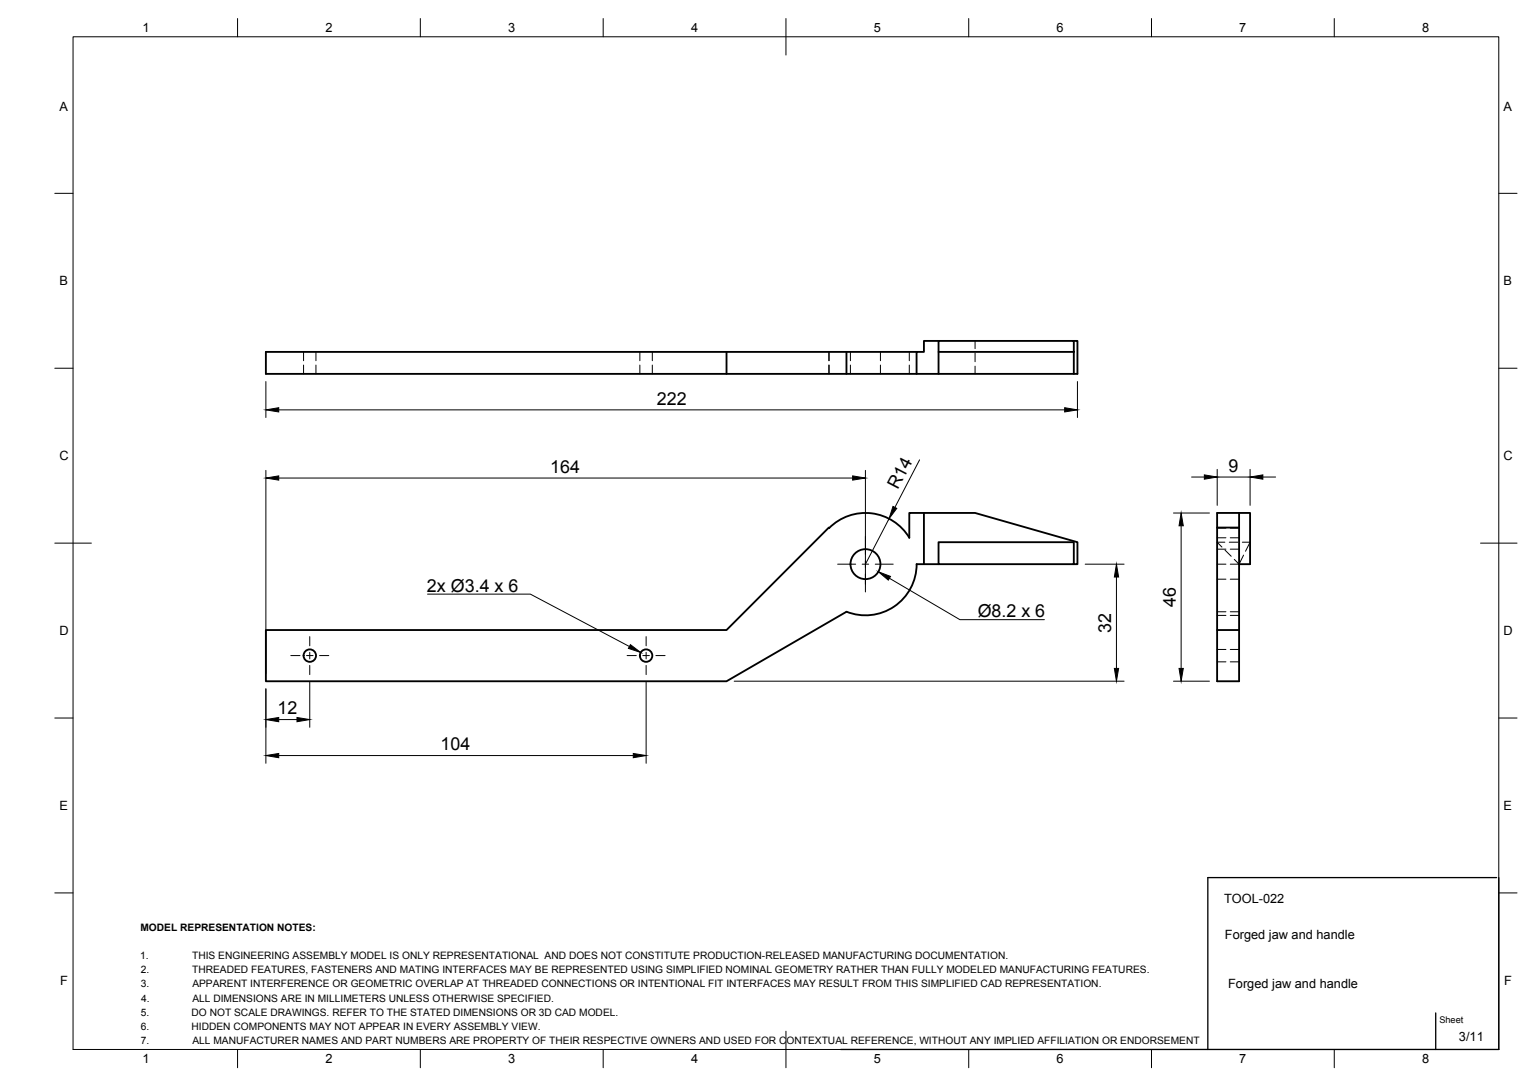
ISO-10303-21;
HEADER;
/* Generated by software containing ST-Developer
 * from STEP Tools, Inc. (www.steptools.com) 
 */

FILE_DESCRIPTION(
/* description */ (''),
/* implementation_level */ '2;1');

FILE_NAME(
/* name */ 'Forged jaw and handle.step',
/* time_stamp */ '2026-11-10T08:27:36-08:00',
/* author */ (''),
/* organization */ (''),
/* preprocessor_version */ 'ST-DEVELOPER v20.2',
/* originating_system */ 'Autodesk Translation Framework v15.17.0.0',
/* authorisation */ '');

FILE_SCHEMA (('AUTOMOTIVE_DESIGN { 1 0 10303 214 3 1 1 }'));
ENDSEC;

DATA;
#10=MECHANICAL_DESIGN_GEOMETRIC_PRESENTATION_REPRESENTATION('',(#566),#19090);
#546=SHAPE_REPRESENTATION_RELATIONSHIP('SRR','None',#19136,#556);
#556=ADVANCED_BREP_SHAPE_REPRESENTATION('',(#576),#19079);
#566=STYLED_ITEM('',(#19200),#576);
#576=MANIFOLD_SOLID_BREP('Body1',#6820);
#586=FACE_BOUND('',#1212,.T.);
#587=FACE_BOUND('',#1213,.T.);
#588=FACE_BOUND('',#1214,.T.);
#589=FACE_BOUND('',#1223,.T.);
#590=FACE_BOUND('',#1224,.T.);
#591=FACE_BOUND('',#1225,.T.);
#653=PLANE('',#6952);
#654=PLANE('',#6953);
#655=PLANE('',#6954);
#656=PLANE('',#6955);
#657=PLANE('',#6956);
#658=PLANE('',#6957);
#659=PLANE('',#6958);
#660=PLANE('',#6959);
#661=PLANE('',#6962);
#662=PLANE('',#6963);
#663=PLANE('',#6964);
#664=PLANE('',#6965);
#665=PLANE('',#6966);
#666=PLANE('',#6967);
#667=PLANE('',#6968);
#668=PLANE('',#6969);
#669=PLANE('',#6973);
#670=PLANE('',#6974);
#671=PLANE('',#6975);
#672=PLANE('',#6976);
#673=PLANE('',#6977);
#674=PLANE('',#6978);
#813=FACE_OUTER_BOUND('',#1201,.T.);
#814=FACE_OUTER_BOUND('',#1202,.T.);
#815=FACE_OUTER_BOUND('',#1203,.T.);
#816=FACE_OUTER_BOUND('',#1204,.T.);
#817=FACE_OUTER_BOUND('',#1205,.T.);
#818=FACE_OUTER_BOUND('',#1206,.T.);
#819=FACE_OUTER_BOUND('',#1207,.T.);
#820=FACE_OUTER_BOUND('',#1208,.T.);
#821=FACE_OUTER_BOUND('',#1209,.T.);
#822=FACE_OUTER_BOUND('',#1210,.T.);
#823=FACE_OUTER_BOUND('',#1211,.T.);
#824=FACE_OUTER_BOUND('',#1215,.T.);
#825=FACE_OUTER_BOUND('',#1216,.T.);
#826=FACE_OUTER_BOUND('',#1217,.T.);
#827=FACE_OUTER_BOUND('',#1218,.T.);
#828=FACE_OUTER_BOUND('',#1219,.T.);
#829=FACE_OUTER_BOUND('',#1220,.T.);
#830=FACE_OUTER_BOUND('',#1221,.T.);
#831=FACE_OUTER_BOUND('',#1222,.T.);
#832=FACE_OUTER_BOUND('',#1226,.T.);
#833=FACE_OUTER_BOUND('',#1227,.T.);
#834=FACE_OUTER_BOUND('',#1228,.T.);
#835=FACE_OUTER_BOUND('',#1229,.T.);
#836=FACE_OUTER_BOUND('',#1230,.T.);
#837=FACE_OUTER_BOUND('',#1231,.T.);
#838=FACE_OUTER_BOUND('',#1232,.T.);
#839=FACE_OUTER_BOUND('',#1233,.T.);
#1201=EDGE_LOOP('',(#4335,#4336,#4337,#4338));
#1202=EDGE_LOOP('',(#4339,#4340,#4341,#4342));
#1203=EDGE_LOOP('',(#4343,#4344,#4345,#4346));
#1204=EDGE_LOOP('',(#4347,#4348,#4349));
#1205=EDGE_LOOP('',(#4350,#4351,#4352,#4353));
#1206=EDGE_LOOP('',(#4354,#4355,#4356));
#1207=EDGE_LOOP('',(#4357,#4358,#4359,#4360,#4361,#4362,#4363));
#1208=EDGE_LOOP('',(#4364,#4365,#4366));
#1209=EDGE_LOOP('',(#4367,#4368,#4369,#4370));
#1210=EDGE_LOOP('',(#4371,#4372,#4373));
#1211=EDGE_LOOP('',(#4374,#4375,#4376,#4377,#4378,#4379,#4380,#4381,#4382,
#4383,#4384,#4385,#4386,#4387,#4388,#4389,#4390));
#1212=EDGE_LOOP('',(#4391));
#1213=EDGE_LOOP('',(#4392));
#1214=EDGE_LOOP('',(#4393));
#1215=EDGE_LOOP('',(#4394,#4395,#4396,#4397));
#1216=EDGE_LOOP('',(#4398,#4399,#4400,#4401,#4402,#4403,#4404,#4405,#4406));
#1217=EDGE_LOOP('',(#4407,#4408,#4409,#4410,#4411));
#1218=EDGE_LOOP('',(#4412,#4413,#4414,#4415));
#1219=EDGE_LOOP('',(#4416,#4417,#4418,#4419));
#1220=EDGE_LOOP('',(#4420,#4421,#4422,#4423));
#1221=EDGE_LOOP('',(#4424,#4425,#4426,#4427,#4428,#4429));
#1222=EDGE_LOOP('',(#4430,#4431,#4432,#4433,#4434,#4435,#4436,#4437,#4438,
#4439,#4440,#4441));
#1223=EDGE_LOOP('',(#4442));
#1224=EDGE_LOOP('',(#4443));
#1225=EDGE_LOOP('',(#4444));
#1226=EDGE_LOOP('',(#4445,#4446,#4447,#4448));
#1227=EDGE_LOOP('',(#4449,#4450,#4451,#4452));
#1228=EDGE_LOOP('',(#4453,#4454,#4455,#4456));
#1229=EDGE_LOOP('',(#4457,#4458,#4459,#4460));
#1230=EDGE_LOOP('',(#4461,#4462,#4463,#4464));
#1231=EDGE_LOOP('',(#4465,#4466,#4467,#4468));
#1232=EDGE_LOOP('',(#4469,#4470,#4471,#4472));
#1233=EDGE_LOOP('',(#4473,#4474,#4475,#4476));
#1656=LINE('',#8884,#2105);
#1657=LINE('',#8890,#2106);
#1658=LINE('',#8896,#2107);
#1659=LINE('',#8901,#2108);
#1660=LINE('',#8903,#2109);
#1661=LINE('',#8904,#2110);
#1662=LINE('',#8908,#2111);
#1663=LINE('',#8909,#2112);
#1664=LINE('',#8910,#2113);
#1665=LINE('',#8913,#2114);
#1666=LINE('',#8914,#2115);
#1667=LINE('',#8917,#2116);
#1668=LINE('',#8919,#2117);
#1669=LINE('',#8921,#2118);
#1670=LINE('',#8923,#2119);
#1671=LINE('',#8925,#2120);
#1672=LINE('',#8926,#2121);
#1673=LINE('',#8929,#2122);
#1674=LINE('',#8930,#2123);
#1675=LINE('',#8933,#2124);
#1676=LINE('',#8934,#2125);
#1677=LINE('',#8937,#2126);
#1678=LINE('',#8938,#2127);
#1679=LINE('',#8943,#2128);
#1680=LINE('',#8945,#2129);
#1681=LINE('',#8947,#2130);
#1682=LINE('',#8949,#2131);
#1683=LINE('',#8951,#2132);
#1684=LINE('',#8953,#2133);
#1685=LINE('',#8957,#2134);
#1686=LINE('',#8959,#2135);
#1687=LINE('',#8961,#2136);
#1688=LINE('',#8963,#2137);
#1689=LINE('',#8964,#2138);
#1690=LINE('',#8967,#2139);
#1691=LINE('',#8969,#2140);
#1692=LINE('',#8970,#2141);
#1693=LINE('',#8973,#2142);
#1694=LINE('',#8975,#2143);
#1695=LINE('',#8977,#2144);
#1696=LINE('',#8978,#2145);
#1697=LINE('',#8980,#2146);
#1698=LINE('',#8983,#2147);
#1699=LINE('',#8985,#2148);
#1700=LINE('',#8986,#2149);
#1701=LINE('',#8988,#2150);
#1702=LINE('',#8990,#2151);
#1703=LINE('',#8992,#2152);
#1704=LINE('',#8997,#2153);
#1705=LINE('',#8999,#2154);
#1706=LINE('',#9001,#2155);
#1707=LINE('',#9003,#2156);
#1708=LINE('',#9005,#2157);
#1709=LINE('',#9007,#2158);
#1710=LINE('',#9010,#2159);
#1711=LINE('',#9012,#2160);
#1712=LINE('',#9013,#2161);
#1713=LINE('',#9015,#2162);
#1714=LINE('',#9017,#2163);
#1715=LINE('',#9019,#2164);
#1716=LINE('',#9021,#2165);
#2105=VECTOR('',#7445,0.17);
#2106=VECTOR('',#7452,0.17);
#2107=VECTOR('',#7459,0.41);
#2108=VECTOR('',#7464,1.);
#2109=VECTOR('',#7465,1.);
#2110=VECTOR('',#7466,1.);
#2111=VECTOR('',#7469,1.);
#2112=VECTOR('',#7470,1.);
#2113=VECTOR('',#7471,1.);
#2114=VECTOR('',#7474,1.);
#2115=VECTOR('',#7475,1.);
#2116=VECTOR('',#7478,1.);
#2117=VECTOR('',#7479,1.);
#2118=VECTOR('',#7480,1.);
#2119=VECTOR('',#7481,1.);
#2120=VECTOR('',#7482,1.);
#2121=VECTOR('',#7483,1.);
#2122=VECTOR('',#7486,1.);
#2123=VECTOR('',#7487,1.);
#2124=VECTOR('',#7490,1.);
#2125=VECTOR('',#7491,1.);
#2126=VECTOR('',#7494,1.);
#2127=VECTOR('',#7495,1.);
#2128=VECTOR('',#7500,1.);
#2129=VECTOR('',#7501,1.);
#2130=VECTOR('',#7502,1.);
#2131=VECTOR('',#7503,1.);
#2132=VECTOR('',#7504,1.);
#2133=VECTOR('',#7505,1.);
#2134=VECTOR('',#7508,1.);
#2135=VECTOR('',#7509,1.);
#2136=VECTOR('',#7510,1.);
#2137=VECTOR('',#7511,1.);
#2138=VECTOR('',#7512,1.);
#2139=VECTOR('',#7515,1.);
#2140=VECTOR('',#7516,1.);
#2141=VECTOR('',#7517,1.);
#2142=VECTOR('',#7520,1.);
#2143=VECTOR('',#7521,1.);
#2144=VECTOR('',#7522,1.);
#2145=VECTOR('',#7523,1.);
#2146=VECTOR('',#7526,1.);
#2147=VECTOR('',#7529,1.);
#2148=VECTOR('',#7530,1.);
#2149=VECTOR('',#7531,1.);
#2150=VECTOR('',#7534,1.);
#2151=VECTOR('',#7537,1.);
#2152=VECTOR('',#7540,1.);
#2153=VECTOR('',#7545,1.);
#2154=VECTOR('',#7546,1.);
#2155=VECTOR('',#7547,1.);
#2156=VECTOR('',#7548,1.);
#2157=VECTOR('',#7549,1.);
#2158=VECTOR('',#7550,1.);
#2159=VECTOR('',#7555,1.);
#2160=VECTOR('',#7558,1.);
#2161=VECTOR('',#7559,1.);
#2162=VECTOR('',#7562,1.);
#2163=VECTOR('',#7565,1.);
#2164=VECTOR('',#7568,1.);
#2165=VECTOR('',#7571,1.);
#2554=CIRCLE('',#6944,0.17);
#2555=CIRCLE('',#6945,0.17);
#2556=CIRCLE('',#6947,0.17);
#2557=CIRCLE('',#6948,0.17);
#2558=CIRCLE('',#6950,0.41);
#2559=CIRCLE('',#6951,0.41);
#2560=CIRCLE('',#6960,1.4);
#2561=CIRCLE('',#6961,1.4);
#2562=CIRCLE('',#6970,1.4);
#2563=CIRCLE('',#6971,1.4);
#2714=VERTEX_POINT('',#8881);
#2715=VERTEX_POINT('',#8883);
#2716=VERTEX_POINT('',#8887);
#2717=VERTEX_POINT('',#8889);
#2718=VERTEX_POINT('',#8893);
#2719=VERTEX_POINT('',#8895);
#2720=VERTEX_POINT('',#8899);
#2721=VERTEX_POINT('',#8900);
#2722=VERTEX_POINT('',#8902);
#2723=VERTEX_POINT('',#8906);
#2724=VERTEX_POINT('',#8907);
#2725=VERTEX_POINT('',#8912);
#2726=VERTEX_POINT('',#8916);
#2727=VERTEX_POINT('',#8918);
#2728=VERTEX_POINT('',#8920);
#2729=VERTEX_POINT('',#8922);
#2730=VERTEX_POINT('',#8924);
#2731=VERTEX_POINT('',#8928);
#2732=VERTEX_POINT('',#8932);
#2733=VERTEX_POINT('',#8936);
#2734=VERTEX_POINT('',#8940);
#2735=VERTEX_POINT('',#8942);
#2736=VERTEX_POINT('',#8944);
#2737=VERTEX_POINT('',#8946);
#2738=VERTEX_POINT('',#8948);
#2739=VERTEX_POINT('',#8950);
#2740=VERTEX_POINT('',#8952);
#2741=VERTEX_POINT('',#8954);
#2742=VERTEX_POINT('',#8956);
#2743=VERTEX_POINT('',#8958);
#2744=VERTEX_POINT('',#8960);
#2745=VERTEX_POINT('',#8962);
#2746=VERTEX_POINT('',#8966);
#2747=VERTEX_POINT('',#8968);
#2748=VERTEX_POINT('',#8972);
#2749=VERTEX_POINT('',#8974);
#2750=VERTEX_POINT('',#8976);
#2751=VERTEX_POINT('',#8982);
#2752=VERTEX_POINT('',#8984);
#2753=VERTEX_POINT('',#8994);
#2754=VERTEX_POINT('',#8996);
#2755=VERTEX_POINT('',#8998);
#2756=VERTEX_POINT('',#9000);
#2757=VERTEX_POINT('',#9002);
#2758=VERTEX_POINT('',#9004);
#2759=VERTEX_POINT('',#9006);
#3352=EDGE_CURVE('',#2714,#2714,#2554,.T.);
#3353=EDGE_CURVE('',#2714,#2715,#1656,.T.);
#3354=EDGE_CURVE('',#2715,#2715,#2555,.T.);
#3355=EDGE_CURVE('',#2716,#2716,#2556,.T.);
#3356=EDGE_CURVE('',#2716,#2717,#1657,.T.);
#3357=EDGE_CURVE('',#2717,#2717,#2557,.T.);
#3358=EDGE_CURVE('',#2718,#2718,#2558,.T.);
#3359=EDGE_CURVE('',#2718,#2719,#1658,.T.);
#3360=EDGE_CURVE('',#2719,#2719,#2559,.T.);
#3361=EDGE_CURVE('',#2720,#2721,#1659,.T.);
#3362=EDGE_CURVE('',#2722,#2720,#1660,.T.);
#3363=EDGE_CURVE('',#2721,#2722,#1661,.T.);
#3364=EDGE_CURVE('',#2723,#2724,#1662,.T.);
#3365=EDGE_CURVE('',#2722,#2723,#1663,.T.);
#3366=EDGE_CURVE('',#2720,#2724,#1664,.T.);
#3367=EDGE_CURVE('',#2725,#2724,#1665,.T.);
#3368=EDGE_CURVE('',#2723,#2725,#1666,.T.);
#3369=EDGE_CURVE('',#2726,#2721,#1667,.T.);
#3370=EDGE_CURVE('',#2726,#2727,#1668,.T.);
#3371=EDGE_CURVE('',#2728,#2727,#1669,.T.);
#3372=EDGE_CURVE('',#2729,#2728,#1670,.T.);
#3373=EDGE_CURVE('',#2730,#2729,#1671,.T.);
#3374=EDGE_CURVE('',#2730,#2720,#1672,.T.);
#3375=EDGE_CURVE('',#2731,#2730,#1673,.T.);
#3376=EDGE_CURVE('',#2720,#2731,#1674,.T.);
#3377=EDGE_CURVE('',#2724,#2732,#1675,.T.);
#3378=EDGE_CURVE('',#2732,#2731,#1676,.T.);
#3379=EDGE_CURVE('',#2733,#2732,#1677,.T.);
#3380=EDGE_CURVE('',#2724,#2733,#1678,.T.);
#3381=EDGE_CURVE('',#2729,#2734,#2560,.T.);
#3382=EDGE_CURVE('',#2734,#2735,#1679,.T.);
#3383=EDGE_CURVE('',#2735,#2736,#1680,.T.);
#3384=EDGE_CURVE('',#2736,#2737,#1681,.T.);
#3385=EDGE_CURVE('',#2737,#2738,#1682,.T.);
#3386=EDGE_CURVE('',#2738,#2739,#1683,.T.);
#3387=EDGE_CURVE('',#2739,#2740,#1684,.T.);
#3388=EDGE_CURVE('',#2740,#2741,#2561,.T.);
#3389=EDGE_CURVE('',#2741,#2742,#1685,.T.);
#3390=EDGE_CURVE('',#2742,#2743,#1686,.T.);
#3391=EDGE_CURVE('',#2743,#2744,#1687,.T.);
#3392=EDGE_CURVE('',#2744,#2745,#1688,.T.);
#3393=EDGE_CURVE('',#2745,#2733,#1689,.T.);
#3394=EDGE_CURVE('',#2746,#2726,#1690,.T.);
#3395=EDGE_CURVE('',#2746,#2747,#1691,.T.);
#3396=EDGE_CURVE('',#2727,#2747,#1692,.T.);
#3397=EDGE_CURVE('',#2725,#2748,#1693,.T.);
#3398=EDGE_CURVE('',#2748,#2749,#1694,.T.);
#3399=EDGE_CURVE('',#2749,#2750,#1695,.T.);
#3400=EDGE_CURVE('',#2750,#2746,#1696,.T.);
#3401=EDGE_CURVE('',#2748,#2745,#1697,.T.);
#3402=EDGE_CURVE('',#2751,#2741,#1698,.T.);
#3403=EDGE_CURVE('',#2752,#2751,#1699,.T.);
#3404=EDGE_CURVE('',#2752,#2742,#1700,.T.);
#3405=EDGE_CURVE('',#2749,#2744,#1701,.T.);
#3406=EDGE_CURVE('',#2750,#2743,#1702,.T.);
#3407=EDGE_CURVE('',#2747,#2752,#1703,.T.);
#3408=EDGE_CURVE('',#2753,#2751,#2562,.T.);
#3409=EDGE_CURVE('',#2754,#2753,#1704,.T.);
#3410=EDGE_CURVE('',#2755,#2754,#1705,.T.);
#3411=EDGE_CURVE('',#2756,#2755,#1706,.T.);
#3412=EDGE_CURVE('',#2757,#2756,#1707,.T.);
#3413=EDGE_CURVE('',#2758,#2757,#1708,.T.);
#3414=EDGE_CURVE('',#2759,#2758,#1709,.T.);
#3415=EDGE_CURVE('',#2728,#2759,#2563,.T.);
#3416=EDGE_CURVE('',#2740,#2753,#1710,.T.);
#3417=EDGE_CURVE('',#2759,#2734,#1711,.T.);
#3418=EDGE_CURVE('',#2758,#2735,#1712,.T.);
#3419=EDGE_CURVE('',#2754,#2739,#1713,.T.);
#3420=EDGE_CURVE('',#2755,#2738,#1714,.T.);
#3421=EDGE_CURVE('',#2756,#2737,#1715,.T.);
#3422=EDGE_CURVE('',#2757,#2736,#1716,.T.);
#4335=ORIENTED_EDGE('',*,*,#3352,.F.);
#4336=ORIENTED_EDGE('',*,*,#3353,.T.);
#4337=ORIENTED_EDGE('',*,*,#3354,.F.);
#4338=ORIENTED_EDGE('',*,*,#3353,.F.);
#4339=ORIENTED_EDGE('',*,*,#3355,.F.);
#4340=ORIENTED_EDGE('',*,*,#3356,.T.);
#4341=ORIENTED_EDGE('',*,*,#3357,.F.);
#4342=ORIENTED_EDGE('',*,*,#3356,.F.);
#4343=ORIENTED_EDGE('',*,*,#3358,.F.);
#4344=ORIENTED_EDGE('',*,*,#3359,.T.);
#4345=ORIENTED_EDGE('',*,*,#3360,.F.);
#4346=ORIENTED_EDGE('',*,*,#3359,.F.);
#4347=ORIENTED_EDGE('',*,*,#3361,.F.);
#4348=ORIENTED_EDGE('',*,*,#3362,.F.);
#4349=ORIENTED_EDGE('',*,*,#3363,.F.);
#4350=ORIENTED_EDGE('',*,*,#3364,.F.);
#4351=ORIENTED_EDGE('',*,*,#3365,.F.);
#4352=ORIENTED_EDGE('',*,*,#3362,.T.);
#4353=ORIENTED_EDGE('',*,*,#3366,.T.);
#4354=ORIENTED_EDGE('',*,*,#3367,.F.);
#4355=ORIENTED_EDGE('',*,*,#3368,.F.);
#4356=ORIENTED_EDGE('',*,*,#3364,.T.);
#4357=ORIENTED_EDGE('',*,*,#3361,.T.);
#4358=ORIENTED_EDGE('',*,*,#3369,.F.);
#4359=ORIENTED_EDGE('',*,*,#3370,.T.);
#4360=ORIENTED_EDGE('',*,*,#3371,.F.);
#4361=ORIENTED_EDGE('',*,*,#3372,.F.);
#4362=ORIENTED_EDGE('',*,*,#3373,.F.);
#4363=ORIENTED_EDGE('',*,*,#3374,.T.);
#4364=ORIENTED_EDGE('',*,*,#3375,.F.);
#4365=ORIENTED_EDGE('',*,*,#3376,.F.);
#4366=ORIENTED_EDGE('',*,*,#3374,.F.);
#4367=ORIENTED_EDGE('',*,*,#3377,.F.);
#4368=ORIENTED_EDGE('',*,*,#3366,.F.);
#4369=ORIENTED_EDGE('',*,*,#3376,.T.);
#4370=ORIENTED_EDGE('',*,*,#3378,.F.);
#4371=ORIENTED_EDGE('',*,*,#3379,.F.);
#4372=ORIENTED_EDGE('',*,*,#3380,.F.);
#4373=ORIENTED_EDGE('',*,*,#3377,.T.);
#4374=ORIENTED_EDGE('',*,*,#3379,.T.);
#4375=ORIENTED_EDGE('',*,*,#3378,.T.);
#4376=ORIENTED_EDGE('',*,*,#3375,.T.);
#4377=ORIENTED_EDGE('',*,*,#3373,.T.);
#4378=ORIENTED_EDGE('',*,*,#3381,.T.);
#4379=ORIENTED_EDGE('',*,*,#3382,.T.);
#4380=ORIENTED_EDGE('',*,*,#3383,.T.);
#4381=ORIENTED_EDGE('',*,*,#3384,.T.);
#4382=ORIENTED_EDGE('',*,*,#3385,.T.);
#4383=ORIENTED_EDGE('',*,*,#3386,.T.);
#4384=ORIENTED_EDGE('',*,*,#3387,.T.);
#4385=ORIENTED_EDGE('',*,*,#3388,.T.);
#4386=ORIENTED_EDGE('',*,*,#3389,.T.);
#4387=ORIENTED_EDGE('',*,*,#3390,.T.);
#4388=ORIENTED_EDGE('',*,*,#3391,.T.);
#4389=ORIENTED_EDGE('',*,*,#3392,.T.);
#4390=ORIENTED_EDGE('',*,*,#3393,.T.);
#4391=ORIENTED_EDGE('',*,*,#3352,.T.);
#4392=ORIENTED_EDGE('',*,*,#3355,.T.);
#4393=ORIENTED_EDGE('',*,*,#3358,.T.);
#4394=ORIENTED_EDGE('',*,*,#3394,.F.);
#4395=ORIENTED_EDGE('',*,*,#3395,.T.);
#4396=ORIENTED_EDGE('',*,*,#3396,.F.);
#4397=ORIENTED_EDGE('',*,*,#3370,.F.);
#4398=ORIENTED_EDGE('',*,*,#3368,.T.);
#4399=ORIENTED_EDGE('',*,*,#3397,.T.);
#4400=ORIENTED_EDGE('',*,*,#3398,.T.);
#4401=ORIENTED_EDGE('',*,*,#3399,.T.);
#4402=ORIENTED_EDGE('',*,*,#3400,.T.);
#4403=ORIENTED_EDGE('',*,*,#3394,.T.);
#4404=ORIENTED_EDGE('',*,*,#3369,.T.);
#4405=ORIENTED_EDGE('',*,*,#3363,.T.);
#4406=ORIENTED_EDGE('',*,*,#3365,.T.);
#4407=ORIENTED_EDGE('',*,*,#3367,.T.);
#4408=ORIENTED_EDGE('',*,*,#3380,.T.);
#4409=ORIENTED_EDGE('',*,*,#3393,.F.);
#4410=ORIENTED_EDGE('',*,*,#3401,.F.);
#4411=ORIENTED_EDGE('',*,*,#3397,.F.);
#4412=ORIENTED_EDGE('',*,*,#3402,.F.);
#4413=ORIENTED_EDGE('',*,*,#3403,.F.);
#4414=ORIENTED_EDGE('',*,*,#3404,.T.);
#4415=ORIENTED_EDGE('',*,*,#3389,.F.);
#4416=ORIENTED_EDGE('',*,*,#3401,.T.);
#4417=ORIENTED_EDGE('',*,*,#3392,.F.);
#4418=ORIENTED_EDGE('',*,*,#3405,.F.);
#4419=ORIENTED_EDGE('',*,*,#3398,.F.);
#4420=ORIENTED_EDGE('',*,*,#3405,.T.);
#4421=ORIENTED_EDGE('',*,*,#3391,.F.);
#4422=ORIENTED_EDGE('',*,*,#3406,.F.);
#4423=ORIENTED_EDGE('',*,*,#3399,.F.);
#4424=ORIENTED_EDGE('',*,*,#3406,.T.);
#4425=ORIENTED_EDGE('',*,*,#3390,.F.);
#4426=ORIENTED_EDGE('',*,*,#3404,.F.);
#4427=ORIENTED_EDGE('',*,*,#3407,.F.);
#4428=ORIENTED_EDGE('',*,*,#3395,.F.);
#4429=ORIENTED_EDGE('',*,*,#3400,.F.);
#4430=ORIENTED_EDGE('',*,*,#3396,.T.);
#4431=ORIENTED_EDGE('',*,*,#3407,.T.);
#4432=ORIENTED_EDGE('',*,*,#3403,.T.);
#4433=ORIENTED_EDGE('',*,*,#3408,.F.);
#4434=ORIENTED_EDGE('',*,*,#3409,.F.);
#4435=ORIENTED_EDGE('',*,*,#3410,.F.);
#4436=ORIENTED_EDGE('',*,*,#3411,.F.);
#4437=ORIENTED_EDGE('',*,*,#3412,.F.);
#4438=ORIENTED_EDGE('',*,*,#3413,.F.);
#4439=ORIENTED_EDGE('',*,*,#3414,.F.);
#4440=ORIENTED_EDGE('',*,*,#3415,.F.);
#4441=ORIENTED_EDGE('',*,*,#3371,.T.);
#4442=ORIENTED_EDGE('',*,*,#3354,.T.);
#4443=ORIENTED_EDGE('',*,*,#3357,.T.);
#4444=ORIENTED_EDGE('',*,*,#3360,.T.);
#4445=ORIENTED_EDGE('',*,*,#3402,.T.);
#4446=ORIENTED_EDGE('',*,*,#3388,.F.);
#4447=ORIENTED_EDGE('',*,*,#3416,.T.);
#4448=ORIENTED_EDGE('',*,*,#3408,.T.);
#4449=ORIENTED_EDGE('',*,*,#3417,.F.);
#4450=ORIENTED_EDGE('',*,*,#3414,.T.);
#4451=ORIENTED_EDGE('',*,*,#3418,.T.);
#4452=ORIENTED_EDGE('',*,*,#3382,.F.);
#4453=ORIENTED_EDGE('',*,*,#3416,.F.);
#4454=ORIENTED_EDGE('',*,*,#3387,.F.);
#4455=ORIENTED_EDGE('',*,*,#3419,.F.);
#4456=ORIENTED_EDGE('',*,*,#3409,.T.);
#4457=ORIENTED_EDGE('',*,*,#3410,.T.);
#4458=ORIENTED_EDGE('',*,*,#3419,.T.);
#4459=ORIENTED_EDGE('',*,*,#3386,.F.);
#4460=ORIENTED_EDGE('',*,*,#3420,.F.);
#4461=ORIENTED_EDGE('',*,*,#3411,.T.);
#4462=ORIENTED_EDGE('',*,*,#3420,.T.);
#4463=ORIENTED_EDGE('',*,*,#3385,.F.);
#4464=ORIENTED_EDGE('',*,*,#3421,.F.);
#4465=ORIENTED_EDGE('',*,*,#3412,.T.);
#4466=ORIENTED_EDGE('',*,*,#3421,.T.);
#4467=ORIENTED_EDGE('',*,*,#3384,.F.);
#4468=ORIENTED_EDGE('',*,*,#3422,.F.);
#4469=ORIENTED_EDGE('',*,*,#3413,.T.);
#4470=ORIENTED_EDGE('',*,*,#3422,.T.);
#4471=ORIENTED_EDGE('',*,*,#3383,.F.);
#4472=ORIENTED_EDGE('',*,*,#3418,.F.);
#4473=ORIENTED_EDGE('',*,*,#3372,.T.);
#4474=ORIENTED_EDGE('',*,*,#3415,.T.);
#4475=ORIENTED_EDGE('',*,*,#3417,.T.);
#4476=ORIENTED_EDGE('',*,*,#3381,.F.);
#6301=CYLINDRICAL_SURFACE('',#6943,0.17);
#6302=CYLINDRICAL_SURFACE('',#6946,0.17);
#6303=CYLINDRICAL_SURFACE('',#6949,0.41);
#6304=CYLINDRICAL_SURFACE('',#6972,1.4);
#6305=CYLINDRICAL_SURFACE('',#6979,1.4);
#6432=ADVANCED_FACE('',(#813),#6301,.F.);
#6433=ADVANCED_FACE('',(#814),#6302,.F.);
#6434=ADVANCED_FACE('',(#815),#6303,.F.);
#6435=ADVANCED_FACE('',(#816),#653,.F.);
#6436=ADVANCED_FACE('',(#817),#654,.F.);
#6437=ADVANCED_FACE('',(#818),#655,.T.);
#6438=ADVANCED_FACE('',(#819),#656,.T.);
#6439=ADVANCED_FACE('',(#820),#657,.F.);
#6440=ADVANCED_FACE('',(#821),#658,.F.);
#6441=ADVANCED_FACE('',(#822),#659,.T.);
#6442=ADVANCED_FACE('',(#823,#586,#587,#588),#660,.T.);
#6443=ADVANCED_FACE('',(#824),#661,.T.);
#6444=ADVANCED_FACE('',(#825),#662,.F.);
#6445=ADVANCED_FACE('',(#826),#663,.T.);
#6446=ADVANCED_FACE('',(#827),#664,.T.);
#6447=ADVANCED_FACE('',(#828),#665,.T.);
#6448=ADVANCED_FACE('',(#829),#666,.T.);
#6449=ADVANCED_FACE('',(#830),#667,.T.);
#6450=ADVANCED_FACE('',(#831,#589,#590,#591),#668,.F.);
#6451=ADVANCED_FACE('',(#832),#6304,.T.);
#6452=ADVANCED_FACE('',(#833),#669,.T.);
#6453=ADVANCED_FACE('',(#834),#670,.T.);
#6454=ADVANCED_FACE('',(#835),#671,.T.);
#6455=ADVANCED_FACE('',(#836),#672,.T.);
#6456=ADVANCED_FACE('',(#837),#673,.T.);
#6457=ADVANCED_FACE('',(#838),#674,.T.);
#6458=ADVANCED_FACE('',(#839),#6305,.T.);
#6820=CLOSED_SHELL('',(#6432,#6433,#6434,#6435,#6436,#6437,#6438,#6439,
#6440,#6441,#6442,#6443,#6444,#6445,#6446,#6447,#6448,#6449,#6450,#6451,
#6452,#6453,#6454,#6455,#6456,#6457,#6458));
#6942=AXIS2_PLACEMENT_3D('',#8879,#7439,#7440);
#6943=AXIS2_PLACEMENT_3D('',#8880,#7441,#7442);
#6944=AXIS2_PLACEMENT_3D('',#8882,#7443,#7444);
#6945=AXIS2_PLACEMENT_3D('',#8885,#7446,#7447);
#6946=AXIS2_PLACEMENT_3D('',#8886,#7448,#7449);
#6947=AXIS2_PLACEMENT_3D('',#8888,#7450,#7451);
#6948=AXIS2_PLACEMENT_3D('',#8891,#7453,#7454);
#6949=AXIS2_PLACEMENT_3D('',#8892,#7455,#7456);
#6950=AXIS2_PLACEMENT_3D('',#8894,#7457,#7458);
#6951=AXIS2_PLACEMENT_3D('',#8897,#7460,#7461);
#6952=AXIS2_PLACEMENT_3D('',#8898,#7462,#7463);
#6953=AXIS2_PLACEMENT_3D('',#8905,#7467,#7468);
#6954=AXIS2_PLACEMENT_3D('',#8911,#7472,#7473);
#6955=AXIS2_PLACEMENT_3D('',#8915,#7476,#7477);
#6956=AXIS2_PLACEMENT_3D('',#8927,#7484,#7485);
#6957=AXIS2_PLACEMENT_3D('',#8931,#7488,#7489);
#6958=AXIS2_PLACEMENT_3D('',#8935,#7492,#7493);
#6959=AXIS2_PLACEMENT_3D('',#8939,#7496,#7497);
#6960=AXIS2_PLACEMENT_3D('',#8941,#7498,#7499);
#6961=AXIS2_PLACEMENT_3D('',#8955,#7506,#7507);
#6962=AXIS2_PLACEMENT_3D('',#8965,#7513,#7514);
#6963=AXIS2_PLACEMENT_3D('',#8971,#7518,#7519);
#6964=AXIS2_PLACEMENT_3D('',#8979,#7524,#7525);
#6965=AXIS2_PLACEMENT_3D('',#8981,#7527,#7528);
#6966=AXIS2_PLACEMENT_3D('',#8987,#7532,#7533);
#6967=AXIS2_PLACEMENT_3D('',#8989,#7535,#7536);
#6968=AXIS2_PLACEMENT_3D('',#8991,#7538,#7539);
#6969=AXIS2_PLACEMENT_3D('',#8993,#7541,#7542);
#6970=AXIS2_PLACEMENT_3D('',#8995,#7543,#7544);
#6971=AXIS2_PLACEMENT_3D('',#9008,#7551,#7552);
#6972=AXIS2_PLACEMENT_3D('',#9009,#7553,#7554);
#6973=AXIS2_PLACEMENT_3D('',#9011,#7556,#7557);
#6974=AXIS2_PLACEMENT_3D('',#9014,#7560,#7561);
#6975=AXIS2_PLACEMENT_3D('',#9016,#7563,#7564);
#6976=AXIS2_PLACEMENT_3D('',#9018,#7566,#7567);
#6977=AXIS2_PLACEMENT_3D('',#9020,#7569,#7570);
#6978=AXIS2_PLACEMENT_3D('',#9022,#7572,#7573);
#6979=AXIS2_PLACEMENT_3D('',#9023,#7574,#7575);
#7439=DIRECTION('axis',(0.,0.,1.));
#7440=DIRECTION('refdir',(1.,0.,0.));
#7441=DIRECTION('center_axis',(0.,0.,-1.));
#7442=DIRECTION('ref_axis',(1.,0.,0.));
#7443=DIRECTION('center_axis',(0.,0.,-1.));
#7444=DIRECTION('ref_axis',(1.,0.,0.));
#7445=DIRECTION('',(0.,0.,-1.));
#7446=DIRECTION('center_axis',(0.,0.,1.));
#7447=DIRECTION('ref_axis',(1.,0.,0.));
#7448=DIRECTION('center_axis',(0.,0.,-1.));
#7449=DIRECTION('ref_axis',(1.,0.,0.));
#7450=DIRECTION('center_axis',(0.,0.,-1.));
#7451=DIRECTION('ref_axis',(1.,0.,0.));
#7452=DIRECTION('',(0.,0.,-1.));
#7453=DIRECTION('center_axis',(0.,0.,1.));
#7454=DIRECTION('ref_axis',(1.,0.,0.));
#7455=DIRECTION('center_axis',(0.,0.,-1.));
#7456=DIRECTION('ref_axis',(1.,0.,0.));
#7457=DIRECTION('center_axis',(0.,0.,-1.));
#7458=DIRECTION('ref_axis',(1.,0.,0.));
#7459=DIRECTION('',(0.,0.,-1.));
#7460=DIRECTION('center_axis',(0.,0.,1.));
#7461=DIRECTION('ref_axis',(1.,0.,0.));
#7462=DIRECTION('center_axis',(1.,0.,0.));
#7463=DIRECTION('ref_axis',(0.,0.,-1.));
#7464=DIRECTION('',(0.,0.,-1.));
#7465=DIRECTION('',(0.,-0.894427190999916,0.447213595499958));
#7466=DIRECTION('',(0.,1.,0.));
#7467=DIRECTION('center_axis',(0.,0.447213595499958,0.894427190999916));
#7468=DIRECTION('ref_axis',(0.,-0.894427190999916,0.447213595499958));
#7469=DIRECTION('',(0.,-0.894427190999916,0.447213595499958));
#7470=DIRECTION('',(-1.,0.,0.));
#7471=DIRECTION('',(-1.,0.,0.));
#7472=DIRECTION('center_axis',(1.,0.,0.));
#7473=DIRECTION('ref_axis',(0.,2.22044604925031E-16,1.));
#7474=DIRECTION('',(0.,0.,1.));
#7475=DIRECTION('',(0.,-1.,0.));
#7476=DIRECTION('center_axis',(0.,-1.,0.));
#7477=DIRECTION('ref_axis',(1.,0.,0.));
#7478=DIRECTION('',(-1.,0.,0.));
#7479=DIRECTION('',(0.,0.,1.));
#7480=DIRECTION('',(-1.,0.,0.));
#7481=DIRECTION('',(0.,0.,-1.));
#7482=DIRECTION('',(1.,0.,0.));
#7483=DIRECTION('',(0.,0.,-1.));
#7484=DIRECTION('center_axis',(1.,0.,0.));
#7485=DIRECTION('ref_axis',(0.,0.,-1.));
#7486=DIRECTION('',(0.,-1.,0.));
#7487=DIRECTION('',(0.,0.707106781186547,0.707106781186548));
#7488=DIRECTION('center_axis',(0.,0.707106781186548,-0.707106781186547));
#7489=DIRECTION('ref_axis',(0.,0.707106781186547,0.707106781186548));
#7490=DIRECTION('',(0.,0.707106781186547,0.707106781186548));
#7491=DIRECTION('',(1.,0.,0.));
#7492=DIRECTION('center_axis',(1.,0.,0.));
#7493=DIRECTION('ref_axis',(0.,2.22044604925031E-16,1.));
#7494=DIRECTION('',(0.,1.,0.));
#7495=DIRECTION('',(0.,0.,1.));
#7496=DIRECTION('center_axis',(0.,0.,1.));
#7497=DIRECTION('ref_axis',(1.,0.,0.));
#7498=DIRECTION('center_axis',(0.,0.,1.));
#7499=DIRECTION('ref_axis',(1.,0.,0.));
#7500=DIRECTION('',(0.865426285481126,-0.501036270541705,0.));
#7501=DIRECTION('',(1.,0.,0.));
#7502=DIRECTION('',(0.,1.,0.));
#7503=DIRECTION('',(-1.,0.,0.));
#7504=DIRECTION('',(-0.707106781186548,0.707106781186548,0.));
#7505=DIRECTION('',(-0.447213595499958,-0.894427190999916,0.));
#7506=DIRECTION('center_axis',(0.,0.,1.));
#7507=DIRECTION('ref_axis',(1.,0.,0.));
#7508=DIRECTION('',(0.,1.,0.));
#7509=DIRECTION('',(-1.,0.,0.));
#7510=DIRECTION('',(-0.961523947640823,-0.274721127897378,0.));
#7511=DIRECTION('',(0.,-1.,0.));
#7512=DIRECTION('',(1.,0.,0.));
#7513=DIRECTION('center_axis',(1.,0.,0.));
#7514=DIRECTION('ref_axis',(0.,1.,0.));
#7515=DIRECTION('',(0.,-1.,0.));
#7516=DIRECTION('',(0.,0.,1.));
#7517=DIRECTION('',(0.,1.,0.));
#7518=DIRECTION('center_axis',(0.,0.,1.));
#7519=DIRECTION('ref_axis',(1.,0.,0.));
#7520=DIRECTION('',(-1.,0.,0.));
#7521=DIRECTION('',(0.,1.,0.));
#7522=DIRECTION('',(0.961523947640823,0.274721127897378,0.));
#7523=DIRECTION('',(1.,0.,0.));
#7524=DIRECTION('center_axis',(0.,-1.,0.));
#7525=DIRECTION('ref_axis',(1.,0.,0.));
#7526=DIRECTION('',(0.,0.,1.));
#7527=DIRECTION('center_axis',(1.,0.,0.));
#7528=DIRECTION('ref_axis',(0.,1.,0.));
#7529=DIRECTION('',(0.,0.,1.));
#7530=DIRECTION('',(0.,-1.,0.));
#7531=DIRECTION('',(0.,0.,1.));
#7532=DIRECTION('center_axis',(-1.,0.,0.));
#7533=DIRECTION('ref_axis',(0.,-1.,0.));
#7534=DIRECTION('',(0.,0.,1.));
#7535=DIRECTION('center_axis',(-0.274721127897378,0.961523947640823,0.));
#7536=DIRECTION('ref_axis',(-0.961523947640823,-0.274721127897378,0.));
#7537=DIRECTION('',(0.,0.,1.));
#7538=DIRECTION('center_axis',(0.,1.,0.));
#7539=DIRECTION('ref_axis',(-1.,0.,0.));
#7540=DIRECTION('',(1.,0.,0.));
#7541=DIRECTION('center_axis',(0.,0.,1.));
#7542=DIRECTION('ref_axis',(1.,0.,0.));
#7543=DIRECTION('center_axis',(0.,0.,1.));
#7544=DIRECTION('ref_axis',(1.,0.,0.));
#7545=DIRECTION('',(-0.447213595499958,-0.894427190999916,0.));
#7546=DIRECTION('',(-0.707106781186548,0.707106781186548,0.));
#7547=DIRECTION('',(-1.,0.,0.));
#7548=DIRECTION('',(0.,1.,0.));
#7549=DIRECTION('',(1.,0.,0.));
#7550=DIRECTION('',(0.865426285481126,-0.501036270541705,0.));
#7551=DIRECTION('center_axis',(0.,0.,1.));
#7552=DIRECTION('ref_axis',(1.,0.,0.));
#7553=DIRECTION('center_axis',(0.,0.,1.));
#7554=DIRECTION('ref_axis',(1.,0.,0.));
#7555=DIRECTION('',(0.,0.,-1.));
#7556=DIRECTION('center_axis',(-0.501036270541705,-0.865426285481126,0.));
#7557=DIRECTION('ref_axis',(0.865426285481126,-0.501036270541705,0.));
#7558=DIRECTION('',(0.,0.,1.));
#7559=DIRECTION('',(0.,0.,1.));
#7560=DIRECTION('center_axis',(-0.894427190999916,0.447213595499958,0.));
#7561=DIRECTION('ref_axis',(-0.447213595499958,-0.894427190999916,0.));
#7562=DIRECTION('',(0.,0.,1.));
#7563=DIRECTION('center_axis',(0.707106781186548,0.707106781186548,0.));
#7564=DIRECTION('ref_axis',(-0.707106781186548,0.707106781186548,0.));
#7565=DIRECTION('',(0.,0.,1.));
#7566=DIRECTION('center_axis',(0.,1.,0.));
#7567=DIRECTION('ref_axis',(-1.,0.,0.));
#7568=DIRECTION('',(0.,0.,1.));
#7569=DIRECTION('center_axis',(1.,0.,0.));
#7570=DIRECTION('ref_axis',(0.,1.,0.));
#7571=DIRECTION('',(0.,0.,1.));
#7572=DIRECTION('center_axis',(0.,-1.,0.));
#7573=DIRECTION('ref_axis',(1.,0.,0.));
#7574=DIRECTION('center_axis',(0.,0.,1.));
#7575=DIRECTION('ref_axis',(1.,0.,0.));
#8879=CARTESIAN_POINT('',(0.,0.,0.));
#8880=CARTESIAN_POINT('Origin',(6.,-2.5,0.3));
#8881=CARTESIAN_POINT('',(5.83,-2.5,0.6));
#8882=CARTESIAN_POINT('Origin',(6.,-2.5,0.6));
#8883=CARTESIAN_POINT('',(5.83,-2.5,0.));
#8884=CARTESIAN_POINT('',(5.83,-2.5,0.3));
#8885=CARTESIAN_POINT('Origin',(6.,-2.5,0.));
#8886=CARTESIAN_POINT('Origin',(15.2,-2.5,0.3));
#8887=CARTESIAN_POINT('',(15.03,-2.5,0.6));
#8888=CARTESIAN_POINT('Origin',(15.2,-2.5,0.6));
#8889=CARTESIAN_POINT('',(15.03,-2.5,0.));
#8890=CARTESIAN_POINT('',(15.03,-2.5,0.3));
#8891=CARTESIAN_POINT('Origin',(15.2,-2.5,0.));
#8892=CARTESIAN_POINT('Origin',(0.,0.,0.3));
#8893=CARTESIAN_POINT('',(-0.41,5.02105187650415E-17,0.6));
#8894=CARTESIAN_POINT('Origin',(0.,0.,0.6));
#8895=CARTESIAN_POINT('',(-0.41,5.02105187650415E-17,0.));
#8896=CARTESIAN_POINT('',(-0.41,5.02105187650415E-17,0.3));
#8897=CARTESIAN_POINT('Origin',(0.,0.,0.));
#8898=CARTESIAN_POINT('Origin',(-2.,0.275,-0.175));
#8899=CARTESIAN_POINT('',(-2.,0.,0.));
#8900=CARTESIAN_POINT('',(-2.,0.,-0.3));
#8901=CARTESIAN_POINT('',(-2.,0.,-0.0875));
#8902=CARTESIAN_POINT('',(-2.,0.6,-0.3));
#8903=CARTESIAN_POINT('',(-2.,0.6,-0.3));
#8904=CARTESIAN_POINT('',(-2.,0.4875,-0.3));
#8905=CARTESIAN_POINT('Origin',(-5.7,0.6,-0.3));
#8906=CARTESIAN_POINT('',(-5.7,0.6,-0.3));
#8907=CARTESIAN_POINT('',(-5.7,0.,0.));
#8908=CARTESIAN_POINT('',(-5.7,0.6,-0.3));
#8909=CARTESIAN_POINT('',(-4.7,0.6,-0.3));
#8910=CARTESIAN_POINT('',(-5.75,0.,0.));
#8911=CARTESIAN_POINT('Origin',(-5.7,0.275,-0.175));
#8912=CARTESIAN_POINT('',(-5.7,0.,-0.3));
#8913=CARTESIAN_POINT('',(-5.7,0.,-0.0875));
#8914=CARTESIAN_POINT('',(-5.7,0.4875,-0.3));
#8915=CARTESIAN_POINT('Origin',(-5.8,0.,0.));
#8916=CARTESIAN_POINT('',(-1.6,0.,-0.3));
#8917=CARTESIAN_POINT('',(-1.6,0.,-0.3));
#8918=CARTESIAN_POINT('',(-1.6,0.,0.));
#8919=CARTESIAN_POINT('',(-1.6,0.,-0.3));
#8920=CARTESIAN_POINT('',(-1.4,0.,0.));
#8921=CARTESIAN_POINT('',(-1.2,0.,0.));
#8922=CARTESIAN_POINT('',(-1.4,0.,0.6));
#8923=CARTESIAN_POINT('',(-1.4,0.,0.));
#8924=CARTESIAN_POINT('',(-2.,0.,0.6));
#8925=CARTESIAN_POINT('',(-1.2,0.,0.6));
#8926=CARTESIAN_POINT('',(-2.,0.,0.1625));
#8927=CARTESIAN_POINT('Origin',(-2.,0.275,0.325));
#8928=CARTESIAN_POINT('',(-2.,0.6,0.6));
#8929=CARTESIAN_POINT('',(-2.,0.1375,0.6));
#8930=CARTESIAN_POINT('',(-2.,0.,0.));
#8931=CARTESIAN_POINT('Origin',(-5.7,0.,0.));
#8932=CARTESIAN_POINT('',(-5.7,0.6,0.6));
#8933=CARTESIAN_POINT('',(-5.7,0.,0.));
#8934=CARTESIAN_POINT('',(-2.85,0.6,0.6));
#8935=CARTESIAN_POINT('Origin',(-5.7,0.275,0.325));
#8936=CARTESIAN_POINT('',(-5.7,0.,0.6));
#8937=CARTESIAN_POINT('',(-5.7,0.1375,0.6));
#8938=CARTESIAN_POINT('',(-5.7,0.,0.1625));
#8939=CARTESIAN_POINT('Origin',(0.,0.,0.6));
#8940=CARTESIAN_POINT('',(0.518766934059614,-1.30033875129767,0.6));
#8941=CARTESIAN_POINT('Origin',(0.,0.,0.6));
#8942=CARTESIAN_POINT('',(3.8,-3.2,0.6));
#8943=CARTESIAN_POINT('',(0.,-1.,0.6));
#8944=CARTESIAN_POINT('',(16.4,-3.2,0.6));
#8945=CARTESIAN_POINT('',(3.8,-3.2,0.6));
#8946=CARTESIAN_POINT('',(16.4,-1.8,0.6));
#8947=CARTESIAN_POINT('',(16.4,-3.2,0.6));
#8948=CARTESIAN_POINT('',(3.8,-1.8,0.6));
#8949=CARTESIAN_POINT('',(16.4,-1.8,0.6));
#8950=CARTESIAN_POINT('',(1.,1.,0.6));
#8951=CARTESIAN_POINT('',(3.8,-1.8,0.6));
#8952=CARTESIAN_POINT('',(0.993295878967653,0.986591757935306,0.6));
#8953=CARTESIAN_POINT('',(1.,1.,0.6));
#8954=CARTESIAN_POINT('',(-1.2,0.721110255092798,0.6));
#8955=CARTESIAN_POINT('Origin',(0.,0.,0.6));
#8956=CARTESIAN_POINT('',(-1.2,1.4,0.6));
#8957=CARTESIAN_POINT('',(-1.2,1.4,0.6));
#8958=CARTESIAN_POINT('',(-3.,1.4,0.6));
#8959=CARTESIAN_POINT('',(-3.,1.4,0.6));
#8960=CARTESIAN_POINT('',(-5.8,0.6,0.6));
#8961=CARTESIAN_POINT('',(-5.8,0.6,0.6));
#8962=CARTESIAN_POINT('',(-5.8,0.,0.6));
#8963=CARTESIAN_POINT('',(-5.8,0.,0.6));
#8964=CARTESIAN_POINT('',(-1.2,0.,0.6));
#8965=CARTESIAN_POINT('Origin',(-1.6,0.,-0.3));
#8966=CARTESIAN_POINT('',(-1.6,1.4,-0.3));
#8967=CARTESIAN_POINT('',(-1.6,1.4,-0.3));
#8968=CARTESIAN_POINT('',(-1.6,1.4,0.));
#8969=CARTESIAN_POINT('',(-1.6,1.4,-0.3));
#8970=CARTESIAN_POINT('',(-1.6,0.,0.));
#8971=CARTESIAN_POINT('Origin',(-3.7,0.7,-0.3));
#8972=CARTESIAN_POINT('',(-5.8,0.,-0.3));
#8973=CARTESIAN_POINT('',(-1.6,0.,-0.3));
#8974=CARTESIAN_POINT('',(-5.8,0.6,-0.3));
#8975=CARTESIAN_POINT('',(-5.8,0.,-0.3));
#8976=CARTESIAN_POINT('',(-3.,1.4,-0.3));
#8977=CARTESIAN_POINT('',(-5.8,0.6,-0.3));
#8978=CARTESIAN_POINT('',(-3.,1.4,-0.3));
#8979=CARTESIAN_POINT('Origin',(-5.8,0.,0.));
#8980=CARTESIAN_POINT('',(-5.8,0.,0.));
#8981=CARTESIAN_POINT('Origin',(-1.2,0.,0.));
#8982=CARTESIAN_POINT('',(-1.2,0.721110255092798,0.));
#8983=CARTESIAN_POINT('',(-1.2,0.721110255092798,0.));
#8984=CARTESIAN_POINT('',(-1.2,1.4,0.));
#8985=CARTESIAN_POINT('',(-1.2,1.4,0.));
#8986=CARTESIAN_POINT('',(-1.2,1.4,0.));
#8987=CARTESIAN_POINT('Origin',(-5.8,0.6,0.));
#8988=CARTESIAN_POINT('',(-5.8,0.6,0.));
#8989=CARTESIAN_POINT('Origin',(-3.,1.4,0.));
#8990=CARTESIAN_POINT('',(-3.,1.4,0.));
#8991=CARTESIAN_POINT('Origin',(-1.2,1.4,0.));
#8992=CARTESIAN_POINT('',(-3.,1.4,0.));
#8993=CARTESIAN_POINT('Origin',(0.,0.,0.));
#8994=CARTESIAN_POINT('',(0.993295878967653,0.986591757935306,0.));
#8995=CARTESIAN_POINT('Origin',(0.,0.,0.));
#8996=CARTESIAN_POINT('',(1.,1.,0.));
#8997=CARTESIAN_POINT('',(1.,1.,0.));
#8998=CARTESIAN_POINT('',(3.8,-1.8,0.));
#8999=CARTESIAN_POINT('',(3.8,-1.8,0.));
#9000=CARTESIAN_POINT('',(16.4,-1.8,0.));
#9001=CARTESIAN_POINT('',(16.4,-1.8,0.));
#9002=CARTESIAN_POINT('',(16.4,-3.2,0.));
#9003=CARTESIAN_POINT('',(16.4,-3.2,0.));
#9004=CARTESIAN_POINT('',(3.8,-3.2,0.));
#9005=CARTESIAN_POINT('',(3.8,-3.2,0.));
#9006=CARTESIAN_POINT('',(0.518766934059614,-1.30033875129767,0.));
#9007=CARTESIAN_POINT('',(0.,-1.,0.));
#9008=CARTESIAN_POINT('Origin',(0.,0.,0.));
#9009=CARTESIAN_POINT('Origin',(0.,0.,0.));
#9010=CARTESIAN_POINT('',(0.993295878967653,0.986591757935306,0.));
#9011=CARTESIAN_POINT('Origin',(0.,-1.,0.));
#9012=CARTESIAN_POINT('',(0.518766934059614,-1.30033875129767,0.));
#9013=CARTESIAN_POINT('',(3.8,-3.2,0.));
#9014=CARTESIAN_POINT('Origin',(1.,1.,0.));
#9015=CARTESIAN_POINT('',(1.,1.,0.));
#9016=CARTESIAN_POINT('Origin',(3.8,-1.8,0.));
#9017=CARTESIAN_POINT('',(3.8,-1.8,0.));
#9018=CARTESIAN_POINT('Origin',(16.4,-1.8,0.));
#9019=CARTESIAN_POINT('',(16.4,-1.8,0.));
#9020=CARTESIAN_POINT('Origin',(16.4,-3.2,0.));
#9021=CARTESIAN_POINT('',(16.4,-3.2,0.));
#9022=CARTESIAN_POINT('Origin',(3.8,-3.2,0.));
#9023=CARTESIAN_POINT('Origin',(0.,0.,0.));
#19066=UNCERTAINTY_MEASURE_WITH_UNIT(LENGTH_MEASURE(0.001),#19091,
'DISTANCE_ACCURACY_VALUE',
'Maximum model space distance between geometric entities at asserted c
onnectivities');
#19077=UNCERTAINTY_MEASURE_WITH_UNIT(LENGTH_MEASURE(0.001),#19091,
'DISTANCE_ACCURACY_VALUE',
'Maximum model space distance between geometric entities at asserted c
onnectivities');
#19079=(
GEOMETRIC_REPRESENTATION_CONTEXT(3)
GLOBAL_UNCERTAINTY_ASSIGNED_CONTEXT((#19066))
GLOBAL_UNIT_ASSIGNED_CONTEXT((#19091,#19093,#19094))
REPRESENTATION_CONTEXT('','3D')
);
#19090=(
GEOMETRIC_REPRESENTATION_CONTEXT(3)
GLOBAL_UNCERTAINTY_ASSIGNED_CONTEXT((#19077))
GLOBAL_UNIT_ASSIGNED_CONTEXT((#19091,#19093,#19094))
REPRESENTATION_CONTEXT('','3D')
);
#19091=(
LENGTH_UNIT()
NAMED_UNIT(*)
SI_UNIT(.CENTI.,.METRE.)
);
#19093=(
NAMED_UNIT(*)
PLANE_ANGLE_UNIT()
SI_UNIT($,.RADIAN.)
);
#19094=(
NAMED_UNIT(*)
SI_UNIT($,.STERADIAN.)
SOLID_ANGLE_UNIT()
);
#19096=SHAPE_DEFINITION_REPRESENTATION(#19108,#19136);
#19108=PRODUCT_DEFINITION_SHAPE('',$,#19149);
#19136=SHAPE_REPRESENTATION('',(#6942),#19079);
#19147=PRODUCT_DEFINITION_CONTEXT('part definition',#19185,'design');
#19149=PRODUCT_DEFINITION('Forged jaw and handle',
'Forged jaw and handle',#19161,#19147);
#19161=PRODUCT_DEFINITION_FORMATION('',$,#19188);
#19185=APPLICATION_CONTEXT(
'Core Data for Automotive Mechanical Design Process');
#19186=PRODUCT_CONTEXT('part definition',#19185,'mechanical');
#19188=PRODUCT('Forged jaw and handle','Forged jaw and handle',$,(#19186));
#19200=PRESENTATION_STYLE_ASSIGNMENT((#19208));
#19208=SURFACE_STYLE_USAGE(.BOTH.,#19216);
#19216=SURFACE_SIDE_STYLE('',(#19224));
#19224=SURFACE_STYLE_FILL_AREA(#19232);
#19232=FILL_AREA_STYLE('Tool steel gray',(#19240));
#19240=FILL_AREA_STYLE_COLOUR('Tool steel gray',#19248);
#19248=COLOUR_RGB('Tool steel gray',0.607843137254902,0.643137254901961,
0.698039215686274);
ENDSEC;
END-ISO-10303-21;
